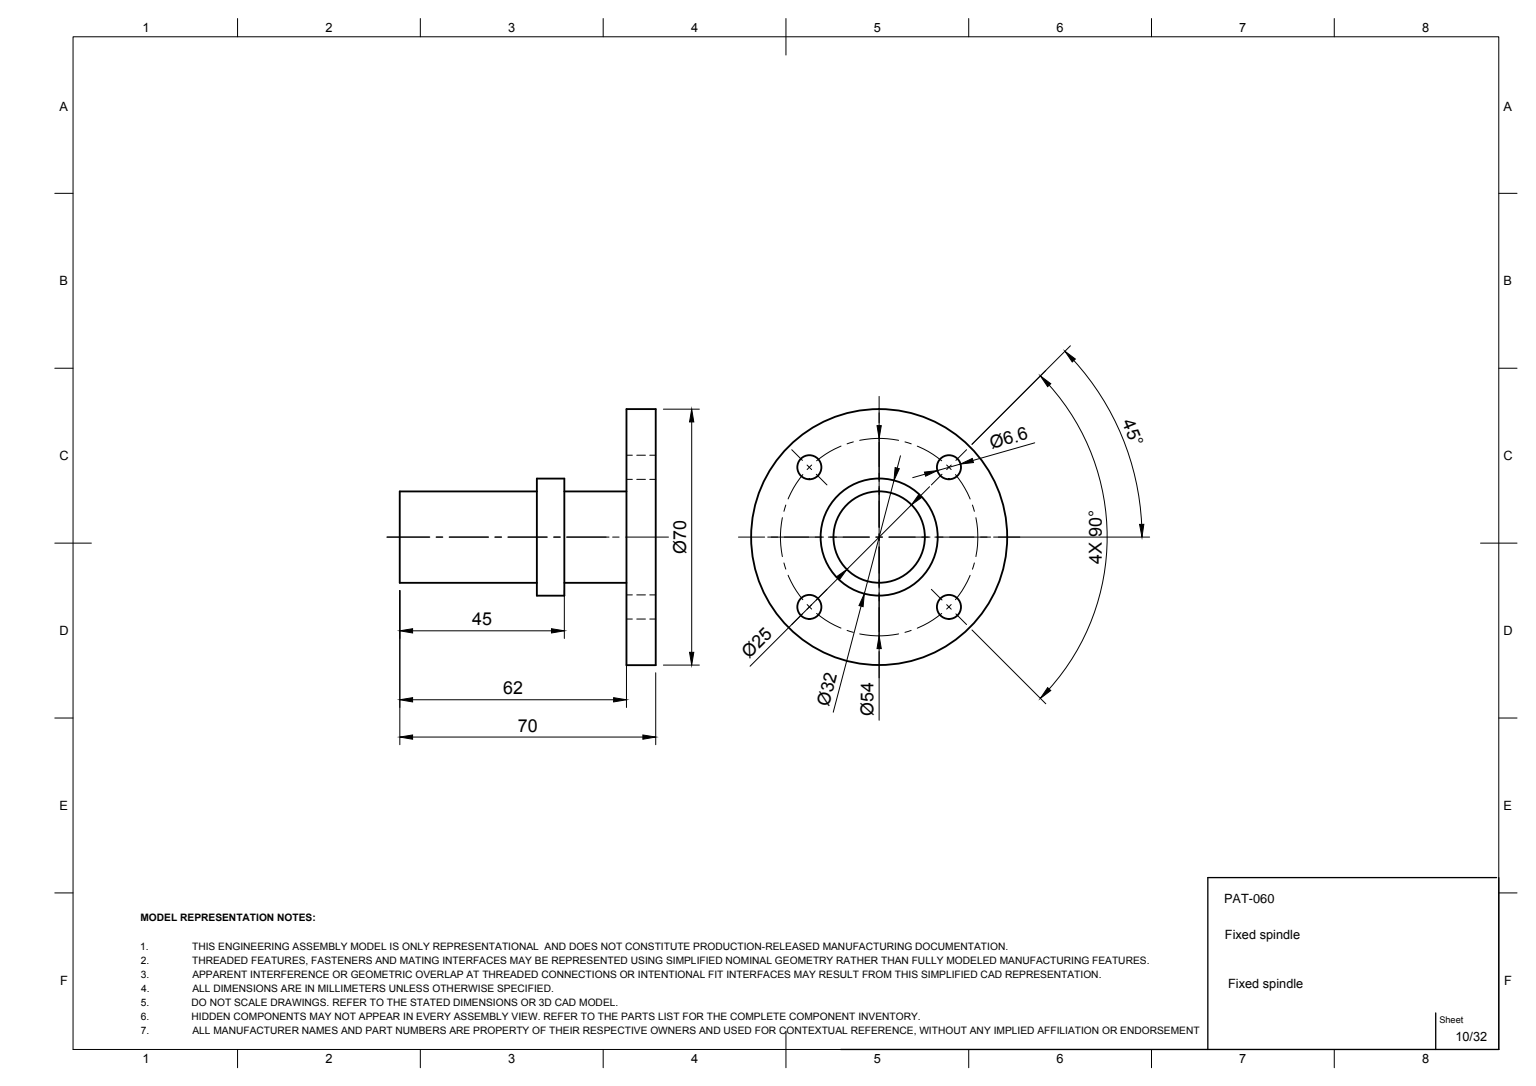
ISO-10303-21;
HEADER;
/* Generated by software containing ST-Developer
 * from STEP Tools, Inc. (www.steptools.com) 
 */

FILE_DESCRIPTION(
/* description */ ('Indexing fixture plate with plunger'),
/* implementation_level */ '2;1');

FILE_NAME(
/* name */ 'Fixed spindle.step',
/* time_stamp */ '2026-10-28T03:23:41-07:00',
/* author */ (''),
/* organization */ (''),
/* preprocessor_version */ 'ST-DEVELOPER v20.2',
/* originating_system */ 'Autodesk Translation Framework v15.17.0.0',
/* authorisation */ '');

FILE_SCHEMA (('AUTOMOTIVE_DESIGN { 1 0 10303 214 3 1 1 }'));
ENDSEC;

DATA;
#10=MECHANICAL_DESIGN_GEOMETRIC_PRESENTATION_REPRESENTATION('',(#322),#10020);
#268=SHAPE_REPRESENTATION_RELATIONSHIP('SRR','None',#10142,#295);
#295=ADVANCED_BREP_SHAPE_REPRESENTATION('',(#358),#9995);
#322=STYLED_ITEM('',(#10361),#358);
#358=MANIFOLD_SOLID_BREP('Body1',#4576);
#401=FACE_BOUND('',#1000,.T.);
#402=FACE_BOUND('',#1002,.T.);
#403=FACE_BOUND('',#1006,.T.);
#404=FACE_BOUND('',#1007,.T.);
#405=FACE_BOUND('',#1008,.T.);
#406=FACE_BOUND('',#1009,.T.);
#407=FACE_BOUND('',#1010,.T.);
#408=FACE_BOUND('',#1015,.T.);
#409=FACE_BOUND('',#1016,.T.);
#410=FACE_BOUND('',#1017,.T.);
#411=FACE_BOUND('',#1018,.T.);
#551=PLANE('',#4974);
#552=PLANE('',#4977);
#553=PLANE('',#4983);
#554=PLANE('',#4989);
#555=PLANE('',#4990);
#695=FACE_OUTER_BOUND('',#995,.T.);
#696=FACE_OUTER_BOUND('',#996,.T.);
#697=FACE_OUTER_BOUND('',#997,.T.);
#698=FACE_OUTER_BOUND('',#998,.T.);
#699=FACE_OUTER_BOUND('',#999,.T.);
#700=FACE_OUTER_BOUND('',#1001,.T.);
#701=FACE_OUTER_BOUND('',#1003,.T.);
#702=FACE_OUTER_BOUND('',#1004,.T.);
#703=FACE_OUTER_BOUND('',#1005,.T.);
#704=FACE_OUTER_BOUND('',#1011,.T.);
#705=FACE_OUTER_BOUND('',#1012,.T.);
#706=FACE_OUTER_BOUND('',#1013,.T.);
#707=FACE_OUTER_BOUND('',#1014,.T.);
#995=EDGE_LOOP('',(#3153,#3154,#3155,#3156));
#996=EDGE_LOOP('',(#3157,#3158,#3159,#3160));
#997=EDGE_LOOP('',(#3161,#3162,#3163,#3164));
#998=EDGE_LOOP('',(#3165,#3166,#3167,#3168));
#999=EDGE_LOOP('',(#3169));
#1000=EDGE_LOOP('',(#3170));
#1001=EDGE_LOOP('',(#3171));
#1002=EDGE_LOOP('',(#3172));
#1003=EDGE_LOOP('',(#3173,#3174,#3175,#3176));
#1004=EDGE_LOOP('',(#3177,#3178,#3179,#3180));
#1005=EDGE_LOOP('',(#3181));
#1006=EDGE_LOOP('',(#3182));
#1007=EDGE_LOOP('',(#3183));
#1008=EDGE_LOOP('',(#3184));
#1009=EDGE_LOOP('',(#3185));
#1010=EDGE_LOOP('',(#3186));
#1011=EDGE_LOOP('',(#3187,#3188,#3189,#3190));
#1012=EDGE_LOOP('',(#3191,#3192,#3193,#3194));
#1013=EDGE_LOOP('',(#3195));
#1014=EDGE_LOOP('',(#3196));
#1015=EDGE_LOOP('',(#3197));
#1016=EDGE_LOOP('',(#3198));
#1017=EDGE_LOOP('',(#3199));
#1018=EDGE_LOOP('',(#3200));
#1415=LINE('',#7237,#1635);
#1416=LINE('',#7243,#1636);
#1417=LINE('',#7249,#1637);
#1418=LINE('',#7255,#1638);
#1419=LINE('',#7268,#1639);
#1420=LINE('',#7271,#1640);
#1421=LINE('',#7278,#1641);
#1422=LINE('',#7283,#1642);
#1635=VECTOR('',#5710,0.33);
#1636=VECTOR('',#5717,0.33);
#1637=VECTOR('',#5724,0.33);
#1638=VECTOR('',#5731,0.33);
#1639=VECTOR('',#5748,1.6);
#1640=VECTOR('',#5751,1.25);
#1641=VECTOR('',#5760,3.5);
#1642=VECTOR('',#5767,1.25);
#1854=CIRCLE('',#4963,0.33);
#1855=CIRCLE('',#4964,0.33);
#1856=CIRCLE('',#4966,0.33);
#1857=CIRCLE('',#4967,0.33);
#1858=CIRCLE('',#4969,0.33);
#1859=CIRCLE('',#4970,0.33);
#1860=CIRCLE('',#4972,0.33);
#1861=CIRCLE('',#4973,0.33);
#1862=CIRCLE('',#4975,1.6);
#1863=CIRCLE('',#4976,1.25);
#1864=CIRCLE('',#4978,1.6);
#1865=CIRCLE('',#4979,1.25);
#1866=CIRCLE('',#4982,1.25);
#1867=CIRCLE('',#4984,3.5);
#1868=CIRCLE('',#4986,3.5);
#1869=CIRCLE('',#4988,1.25);
#2165=VERTEX_POINT('',#7234);
#2166=VERTEX_POINT('',#7236);
#2167=VERTEX_POINT('',#7240);
#2168=VERTEX_POINT('',#7242);
#2169=VERTEX_POINT('',#7246);
#2170=VERTEX_POINT('',#7248);
#2171=VERTEX_POINT('',#7252);
#2172=VERTEX_POINT('',#7254);
#2173=VERTEX_POINT('',#7258);
#2174=VERTEX_POINT('',#7260);
#2175=VERTEX_POINT('',#7263);
#2176=VERTEX_POINT('',#7265);
#2177=VERTEX_POINT('',#7270);
#2178=VERTEX_POINT('',#7274);
#2179=VERTEX_POINT('',#7277);
#2180=VERTEX_POINT('',#7281);
#2556=EDGE_CURVE('',#2165,#2165,#1854,.T.);
#2557=EDGE_CURVE('',#2165,#2166,#1415,.T.);
#2558=EDGE_CURVE('',#2166,#2166,#1855,.T.);
#2559=EDGE_CURVE('',#2167,#2167,#1856,.T.);
#2560=EDGE_CURVE('',#2167,#2168,#1416,.T.);
#2561=EDGE_CURVE('',#2168,#2168,#1857,.T.);
#2562=EDGE_CURVE('',#2169,#2169,#1858,.T.);
#2563=EDGE_CURVE('',#2169,#2170,#1417,.T.);
#2564=EDGE_CURVE('',#2170,#2170,#1859,.T.);
#2565=EDGE_CURVE('',#2171,#2171,#1860,.T.);
#2566=EDGE_CURVE('',#2171,#2172,#1418,.T.);
#2567=EDGE_CURVE('',#2172,#2172,#1861,.T.);
#2568=EDGE_CURVE('',#2173,#2173,#1862,.T.);
#2569=EDGE_CURVE('',#2174,#2174,#1863,.T.);
#2570=EDGE_CURVE('',#2175,#2175,#1864,.T.);
#2571=EDGE_CURVE('',#2176,#2176,#1865,.T.);
#2572=EDGE_CURVE('',#2173,#2175,#1419,.T.);
#2573=EDGE_CURVE('',#2176,#2177,#1420,.T.);
#2574=EDGE_CURVE('',#2177,#2177,#1866,.T.);
#2575=EDGE_CURVE('',#2178,#2178,#1867,.T.);
#2576=EDGE_CURVE('',#2178,#2179,#1421,.T.);
#2577=EDGE_CURVE('',#2179,#2179,#1868,.T.);
#2578=EDGE_CURVE('',#2180,#2180,#1869,.T.);
#2579=EDGE_CURVE('',#2180,#2174,#1422,.T.);
#3153=ORIENTED_EDGE('',*,*,#2556,.F.);
#3154=ORIENTED_EDGE('',*,*,#2557,.T.);
#3155=ORIENTED_EDGE('',*,*,#2558,.F.);
#3156=ORIENTED_EDGE('',*,*,#2557,.F.);
#3157=ORIENTED_EDGE('',*,*,#2559,.F.);
#3158=ORIENTED_EDGE('',*,*,#2560,.T.);
#3159=ORIENTED_EDGE('',*,*,#2561,.F.);
#3160=ORIENTED_EDGE('',*,*,#2560,.F.);
#3161=ORIENTED_EDGE('',*,*,#2562,.F.);
#3162=ORIENTED_EDGE('',*,*,#2563,.T.);
#3163=ORIENTED_EDGE('',*,*,#2564,.F.);
#3164=ORIENTED_EDGE('',*,*,#2563,.F.);
#3165=ORIENTED_EDGE('',*,*,#2565,.F.);
#3166=ORIENTED_EDGE('',*,*,#2566,.T.);
#3167=ORIENTED_EDGE('',*,*,#2567,.F.);
#3168=ORIENTED_EDGE('',*,*,#2566,.F.);
#3169=ORIENTED_EDGE('',*,*,#2568,.T.);
#3170=ORIENTED_EDGE('',*,*,#2569,.F.);
#3171=ORIENTED_EDGE('',*,*,#2570,.F.);
#3172=ORIENTED_EDGE('',*,*,#2571,.F.);
#3173=ORIENTED_EDGE('',*,*,#2568,.F.);
#3174=ORIENTED_EDGE('',*,*,#2572,.T.);
#3175=ORIENTED_EDGE('',*,*,#2570,.T.);
#3176=ORIENTED_EDGE('',*,*,#2572,.F.);
#3177=ORIENTED_EDGE('',*,*,#2571,.T.);
#3178=ORIENTED_EDGE('',*,*,#2573,.T.);
#3179=ORIENTED_EDGE('',*,*,#2574,.T.);
#3180=ORIENTED_EDGE('',*,*,#2573,.F.);
#3181=ORIENTED_EDGE('',*,*,#2575,.T.);
#3182=ORIENTED_EDGE('',*,*,#2574,.F.);
#3183=ORIENTED_EDGE('',*,*,#2567,.T.);
#3184=ORIENTED_EDGE('',*,*,#2564,.T.);
#3185=ORIENTED_EDGE('',*,*,#2561,.T.);
#3186=ORIENTED_EDGE('',*,*,#2558,.T.);
#3187=ORIENTED_EDGE('',*,*,#2575,.F.);
#3188=ORIENTED_EDGE('',*,*,#2576,.T.);
#3189=ORIENTED_EDGE('',*,*,#2577,.T.);
#3190=ORIENTED_EDGE('',*,*,#2576,.F.);
#3191=ORIENTED_EDGE('',*,*,#2578,.F.);
#3192=ORIENTED_EDGE('',*,*,#2579,.T.);
#3193=ORIENTED_EDGE('',*,*,#2569,.T.);
#3194=ORIENTED_EDGE('',*,*,#2579,.F.);
#3195=ORIENTED_EDGE('',*,*,#2578,.T.);
#3196=ORIENTED_EDGE('',*,*,#2577,.F.);
#3197=ORIENTED_EDGE('',*,*,#2556,.T.);
#3198=ORIENTED_EDGE('',*,*,#2559,.T.);
#3199=ORIENTED_EDGE('',*,*,#2562,.T.);
#3200=ORIENTED_EDGE('',*,*,#2565,.T.);
#4178=CYLINDRICAL_SURFACE('',#4962,0.33);
#4179=CYLINDRICAL_SURFACE('',#4965,0.33);
#4180=CYLINDRICAL_SURFACE('',#4968,0.33);
#4181=CYLINDRICAL_SURFACE('',#4971,0.33);
#4182=CYLINDRICAL_SURFACE('',#4980,1.6);
#4183=CYLINDRICAL_SURFACE('',#4981,1.25);
#4184=CYLINDRICAL_SURFACE('',#4985,3.5);
#4185=CYLINDRICAL_SURFACE('',#4987,1.25);
#4310=ADVANCED_FACE('',(#695),#4178,.F.);
#4311=ADVANCED_FACE('',(#696),#4179,.F.);
#4312=ADVANCED_FACE('',(#697),#4180,.F.);
#4313=ADVANCED_FACE('',(#698),#4181,.F.);
#4314=ADVANCED_FACE('',(#699,#401),#551,.T.);
#4315=ADVANCED_FACE('',(#700,#402),#552,.F.);
#4316=ADVANCED_FACE('',(#701),#4182,.T.);
#4317=ADVANCED_FACE('',(#702),#4183,.T.);
#4318=ADVANCED_FACE('',(#703,#403,#404,#405,#406,#407),#553,.T.);
#4319=ADVANCED_FACE('',(#704),#4184,.T.);
#4320=ADVANCED_FACE('',(#705),#4185,.T.);
#4321=ADVANCED_FACE('',(#706),#554,.T.);
#4322=ADVANCED_FACE('',(#707,#408,#409,#410,#411),#555,.F.);
#4576=CLOSED_SHELL('',(#4310,#4311,#4312,#4313,#4314,#4315,#4316,#4317,
#4318,#4319,#4320,#4321,#4322));
#4961=AXIS2_PLACEMENT_3D('',#7232,#5704,#5705);
#4962=AXIS2_PLACEMENT_3D('',#7233,#5706,#5707);
#4963=AXIS2_PLACEMENT_3D('',#7235,#5708,#5709);
#4964=AXIS2_PLACEMENT_3D('',#7238,#5711,#5712);
#4965=AXIS2_PLACEMENT_3D('',#7239,#5713,#5714);
#4966=AXIS2_PLACEMENT_3D('',#7241,#5715,#5716);
#4967=AXIS2_PLACEMENT_3D('',#7244,#5718,#5719);
#4968=AXIS2_PLACEMENT_3D('',#7245,#5720,#5721);
#4969=AXIS2_PLACEMENT_3D('',#7247,#5722,#5723);
#4970=AXIS2_PLACEMENT_3D('',#7250,#5725,#5726);
#4971=AXIS2_PLACEMENT_3D('',#7251,#5727,#5728);
#4972=AXIS2_PLACEMENT_3D('',#7253,#5729,#5730);
#4973=AXIS2_PLACEMENT_3D('',#7256,#5732,#5733);
#4974=AXIS2_PLACEMENT_3D('',#7257,#5734,#5735);
#4975=AXIS2_PLACEMENT_3D('',#7259,#5736,#5737);
#4976=AXIS2_PLACEMENT_3D('',#7261,#5738,#5739);
#4977=AXIS2_PLACEMENT_3D('',#7262,#5740,#5741);
#4978=AXIS2_PLACEMENT_3D('',#7264,#5742,#5743);
#4979=AXIS2_PLACEMENT_3D('',#7266,#5744,#5745);
#4980=AXIS2_PLACEMENT_3D('',#7267,#5746,#5747);
#4981=AXIS2_PLACEMENT_3D('',#7269,#5749,#5750);
#4982=AXIS2_PLACEMENT_3D('',#7272,#5752,#5753);
#4983=AXIS2_PLACEMENT_3D('',#7273,#5754,#5755);
#4984=AXIS2_PLACEMENT_3D('',#7275,#5756,#5757);
#4985=AXIS2_PLACEMENT_3D('',#7276,#5758,#5759);
#4986=AXIS2_PLACEMENT_3D('',#7279,#5761,#5762);
#4987=AXIS2_PLACEMENT_3D('',#7280,#5763,#5764);
#4988=AXIS2_PLACEMENT_3D('',#7282,#5765,#5766);
#4989=AXIS2_PLACEMENT_3D('',#7284,#5768,#5769);
#4990=AXIS2_PLACEMENT_3D('',#7285,#5770,#5771);
#5704=DIRECTION('axis',(0.,0.,1.));
#5705=DIRECTION('refdir',(1.,0.,0.));
#5706=DIRECTION('center_axis',(0.,0.,1.));
#5707=DIRECTION('ref_axis',(1.,0.,0.));
#5708=DIRECTION('center_axis',(0.,0.,1.));
#5709=DIRECTION('ref_axis',(1.,0.,0.));
#5710=DIRECTION('',(0.,0.,1.));
#5711=DIRECTION('center_axis',(0.,0.,-1.));
#5712=DIRECTION('ref_axis',(1.,0.,0.));
#5713=DIRECTION('center_axis',(0.,0.,1.));
#5714=DIRECTION('ref_axis',(1.,0.,0.));
#5715=DIRECTION('center_axis',(0.,0.,1.));
#5716=DIRECTION('ref_axis',(1.,0.,0.));
#5717=DIRECTION('',(0.,0.,1.));
#5718=DIRECTION('center_axis',(0.,0.,-1.));
#5719=DIRECTION('ref_axis',(1.,0.,0.));
#5720=DIRECTION('center_axis',(0.,0.,1.));
#5721=DIRECTION('ref_axis',(1.,0.,0.));
#5722=DIRECTION('center_axis',(0.,0.,1.));
#5723=DIRECTION('ref_axis',(1.,0.,0.));
#5724=DIRECTION('',(0.,0.,1.));
#5725=DIRECTION('center_axis',(0.,0.,-1.));
#5726=DIRECTION('ref_axis',(1.,0.,0.));
#5727=DIRECTION('center_axis',(0.,0.,1.));
#5728=DIRECTION('ref_axis',(1.,0.,0.));
#5729=DIRECTION('center_axis',(0.,0.,1.));
#5730=DIRECTION('ref_axis',(1.,0.,0.));
#5731=DIRECTION('',(0.,0.,1.));
#5732=DIRECTION('center_axis',(0.,0.,-1.));
#5733=DIRECTION('ref_axis',(1.,0.,0.));
#5734=DIRECTION('center_axis',(0.,0.,1.));
#5735=DIRECTION('ref_axis',(1.,0.,0.));
#5736=DIRECTION('center_axis',(0.,0.,1.));
#5737=DIRECTION('ref_axis',(1.,0.,0.));
#5738=DIRECTION('center_axis',(0.,0.,1.));
#5739=DIRECTION('ref_axis',(1.,0.,0.));
#5740=DIRECTION('center_axis',(0.,0.,1.));
#5741=DIRECTION('ref_axis',(1.,0.,0.));
#5742=DIRECTION('center_axis',(0.,0.,1.));
#5743=DIRECTION('ref_axis',(1.,0.,0.));
#5744=DIRECTION('center_axis',(0.,0.,-1.));
#5745=DIRECTION('ref_axis',(1.,0.,0.));
#5746=DIRECTION('center_axis',(0.,0.,1.));
#5747=DIRECTION('ref_axis',(1.,0.,0.));
#5748=DIRECTION('',(0.,0.,-1.));
#5749=DIRECTION('center_axis',(0.,0.,1.));
#5750=DIRECTION('ref_axis',(1.,0.,0.));
#5751=DIRECTION('',(0.,0.,-1.));
#5752=DIRECTION('center_axis',(0.,0.,1.));
#5753=DIRECTION('ref_axis',(1.,0.,0.));
#5754=DIRECTION('center_axis',(0.,0.,1.));
#5755=DIRECTION('ref_axis',(1.,0.,0.));
#5756=DIRECTION('center_axis',(0.,0.,1.));
#5757=DIRECTION('ref_axis',(1.,0.,0.));
#5758=DIRECTION('center_axis',(0.,0.,1.));
#5759=DIRECTION('ref_axis',(1.,0.,0.));
#5760=DIRECTION('',(0.,0.,-1.));
#5761=DIRECTION('center_axis',(0.,0.,1.));
#5762=DIRECTION('ref_axis',(1.,0.,0.));
#5763=DIRECTION('center_axis',(0.,0.,1.));
#5764=DIRECTION('ref_axis',(1.,0.,0.));
#5765=DIRECTION('center_axis',(0.,0.,1.));
#5766=DIRECTION('ref_axis',(1.,0.,0.));
#5767=DIRECTION('',(0.,0.,-1.));
#5768=DIRECTION('center_axis',(0.,0.,1.));
#5769=DIRECTION('ref_axis',(1.,0.,0.));
#5770=DIRECTION('center_axis',(0.,0.,1.));
#5771=DIRECTION('ref_axis',(1.,0.,0.));
#7232=CARTESIAN_POINT('',(0.,0.,0.));
#7233=CARTESIAN_POINT('Origin',(-1.90918830920368,-1.90918830920368,-0.1));
#7234=CARTESIAN_POINT('',(-2.23918830920368,-1.90918830920368,0.));
#7235=CARTESIAN_POINT('Origin',(-1.90918830920368,-1.90918830920368,0.));
#7236=CARTESIAN_POINT('',(-2.23918830920368,-1.90918830920368,0.8));
#7237=CARTESIAN_POINT('',(-2.23918830920368,-1.90918830920368,-0.1));
#7238=CARTESIAN_POINT('Origin',(-1.90918830920368,-1.90918830920368,0.8));
#7239=CARTESIAN_POINT('Origin',(-1.90918830920368,1.90918830920368,-0.1));
#7240=CARTESIAN_POINT('',(-2.23918830920368,1.90918830920368,0.));
#7241=CARTESIAN_POINT('Origin',(-1.90918830920368,1.90918830920368,0.));
#7242=CARTESIAN_POINT('',(-2.23918830920368,1.90918830920368,0.8));
#7243=CARTESIAN_POINT('',(-2.23918830920368,1.90918830920368,-0.1));
#7244=CARTESIAN_POINT('Origin',(-1.90918830920368,1.90918830920368,0.8));
#7245=CARTESIAN_POINT('Origin',(1.90918830920368,1.90918830920368,-0.1));
#7246=CARTESIAN_POINT('',(1.57918830920368,1.90918830920368,0.));
#7247=CARTESIAN_POINT('Origin',(1.90918830920368,1.90918830920368,0.));
#7248=CARTESIAN_POINT('',(1.57918830920368,1.90918830920368,0.8));
#7249=CARTESIAN_POINT('',(1.57918830920368,1.90918830920368,-0.1));
#7250=CARTESIAN_POINT('Origin',(1.90918830920368,1.90918830920368,0.8));
#7251=CARTESIAN_POINT('Origin',(1.90918830920368,-1.90918830920368,-0.1));
#7252=CARTESIAN_POINT('',(1.57918830920368,-1.90918830920368,0.));
#7253=CARTESIAN_POINT('Origin',(1.90918830920368,-1.90918830920368,0.));
#7254=CARTESIAN_POINT('',(1.57918830920368,-1.90918830920368,0.8));
#7255=CARTESIAN_POINT('',(1.57918830920368,-1.90918830920368,-0.1));
#7256=CARTESIAN_POINT('Origin',(1.90918830920368,-1.90918830920368,0.8));
#7257=CARTESIAN_POINT('Origin',(0.,0.,3.25));
#7258=CARTESIAN_POINT('',(-1.6,-1.95943487863577E-16,3.25));
#7259=CARTESIAN_POINT('Origin',(0.,0.,3.25));
#7260=CARTESIAN_POINT('',(-1.25,-1.53080849893419E-16,3.25));
#7261=CARTESIAN_POINT('Origin',(0.,0.,3.25));
#7262=CARTESIAN_POINT('Origin',(0.,0.,2.5));
#7263=CARTESIAN_POINT('',(-1.6,-1.95943487863577E-16,2.5));
#7264=CARTESIAN_POINT('Origin',(0.,0.,2.5));
#7265=CARTESIAN_POINT('',(-1.25,1.53080849893419E-16,2.5));
#7266=CARTESIAN_POINT('Origin',(0.,0.,2.5));
#7267=CARTESIAN_POINT('Origin',(0.,0.,2.5));
#7268=CARTESIAN_POINT('',(-1.6,-1.95943487863577E-16,2.5));
#7269=CARTESIAN_POINT('Origin',(0.,0.,0.));
#7270=CARTESIAN_POINT('',(-1.25,-1.53080849893419E-16,0.8));
#7271=CARTESIAN_POINT('',(-1.25,-1.53080849893419E-16,0.));
#7272=CARTESIAN_POINT('Origin',(0.,0.,0.8));
#7273=CARTESIAN_POINT('Origin',(0.,0.,0.8));
#7274=CARTESIAN_POINT('',(-3.5,-4.28626379701574E-16,0.8));
#7275=CARTESIAN_POINT('Origin',(0.,0.,0.8));
#7276=CARTESIAN_POINT('Origin',(0.,0.,0.));
#7277=CARTESIAN_POINT('',(-3.5,-4.28626379701574E-16,0.));
#7278=CARTESIAN_POINT('',(-3.5,-4.28626379701574E-16,0.));
#7279=CARTESIAN_POINT('Origin',(0.,0.,0.));
#7280=CARTESIAN_POINT('Origin',(0.,0.,0.));
#7281=CARTESIAN_POINT('',(-1.25,-1.53080849893419E-16,7.));
#7282=CARTESIAN_POINT('Origin',(0.,0.,7.));
#7283=CARTESIAN_POINT('',(-1.25,-1.53080849893419E-16,0.));
#7284=CARTESIAN_POINT('Origin',(0.,0.,7.));
#7285=CARTESIAN_POINT('Origin',(0.,0.,0.));
#9962=UNCERTAINTY_MEASURE_WITH_UNIT(LENGTH_MEASURE(0.001),#10021,
'DISTANCE_ACCURACY_VALUE',
'Maximum model space distance between geometric entities at asserted c
onnectivities');
#9987=UNCERTAINTY_MEASURE_WITH_UNIT(LENGTH_MEASURE(0.001),#10021,
'DISTANCE_ACCURACY_VALUE',
'Maximum model space distance between geometric entities at asserted c
onnectivities');
#9995=(
GEOMETRIC_REPRESENTATION_CONTEXT(3)
GLOBAL_UNCERTAINTY_ASSIGNED_CONTEXT((#9962))
GLOBAL_UNIT_ASSIGNED_CONTEXT((#10021,#10023,#10024))
REPRESENTATION_CONTEXT('','3D')
);
#10020=(
GEOMETRIC_REPRESENTATION_CONTEXT(3)
GLOBAL_UNCERTAINTY_ASSIGNED_CONTEXT((#9987))
GLOBAL_UNIT_ASSIGNED_CONTEXT((#10021,#10023,#10024))
REPRESENTATION_CONTEXT('','3D')
);
#10021=(
LENGTH_UNIT()
NAMED_UNIT(*)
SI_UNIT(.CENTI.,.METRE.)
);
#10023=(
NAMED_UNIT(*)
PLANE_ANGLE_UNIT()
SI_UNIT($,.RADIAN.)
);
#10024=(
NAMED_UNIT(*)
SI_UNIT($,.STERADIAN.)
SOLID_ANGLE_UNIT()
);
#10032=SHAPE_DEFINITION_REPRESENTATION(#10064,#10142);
#10064=PRODUCT_DEFINITION_SHAPE('',$,#10175);
#10142=SHAPE_REPRESENTATION('',(#4961),#9995);
#10167=PRODUCT_DEFINITION_CONTEXT('part definition',#10265,'design');
#10175=PRODUCT_DEFINITION('Fixed spindle','Fixed spindle',#10207,#10167);
#10207=PRODUCT_DEFINITION_FORMATION('',$,#10274);
#10265=APPLICATION_CONTEXT(
'Core Data for Automotive Mechanical Design Process');
#10266=PRODUCT_CONTEXT('part definition',#10265,'mechanical');
#10274=PRODUCT('Fixed spindle','Fixed spindle','Fixed spindle',(#10266));
#10355=COLOUR_RGB('Sky Blue',0.24,0.69,0.87);
#10356=FILL_AREA_STYLE_COLOUR('',#10355);
#10357=FILL_AREA_STYLE('',(#10356));
#10358=SURFACE_STYLE_FILL_AREA(#10357);
#10359=SURFACE_SIDE_STYLE('',(#10358));
#10360=SURFACE_STYLE_USAGE(.BOTH.,#10359);
#10361=PRESENTATION_STYLE_ASSIGNMENT((#10360));
ENDSEC;
END-ISO-10303-21;
